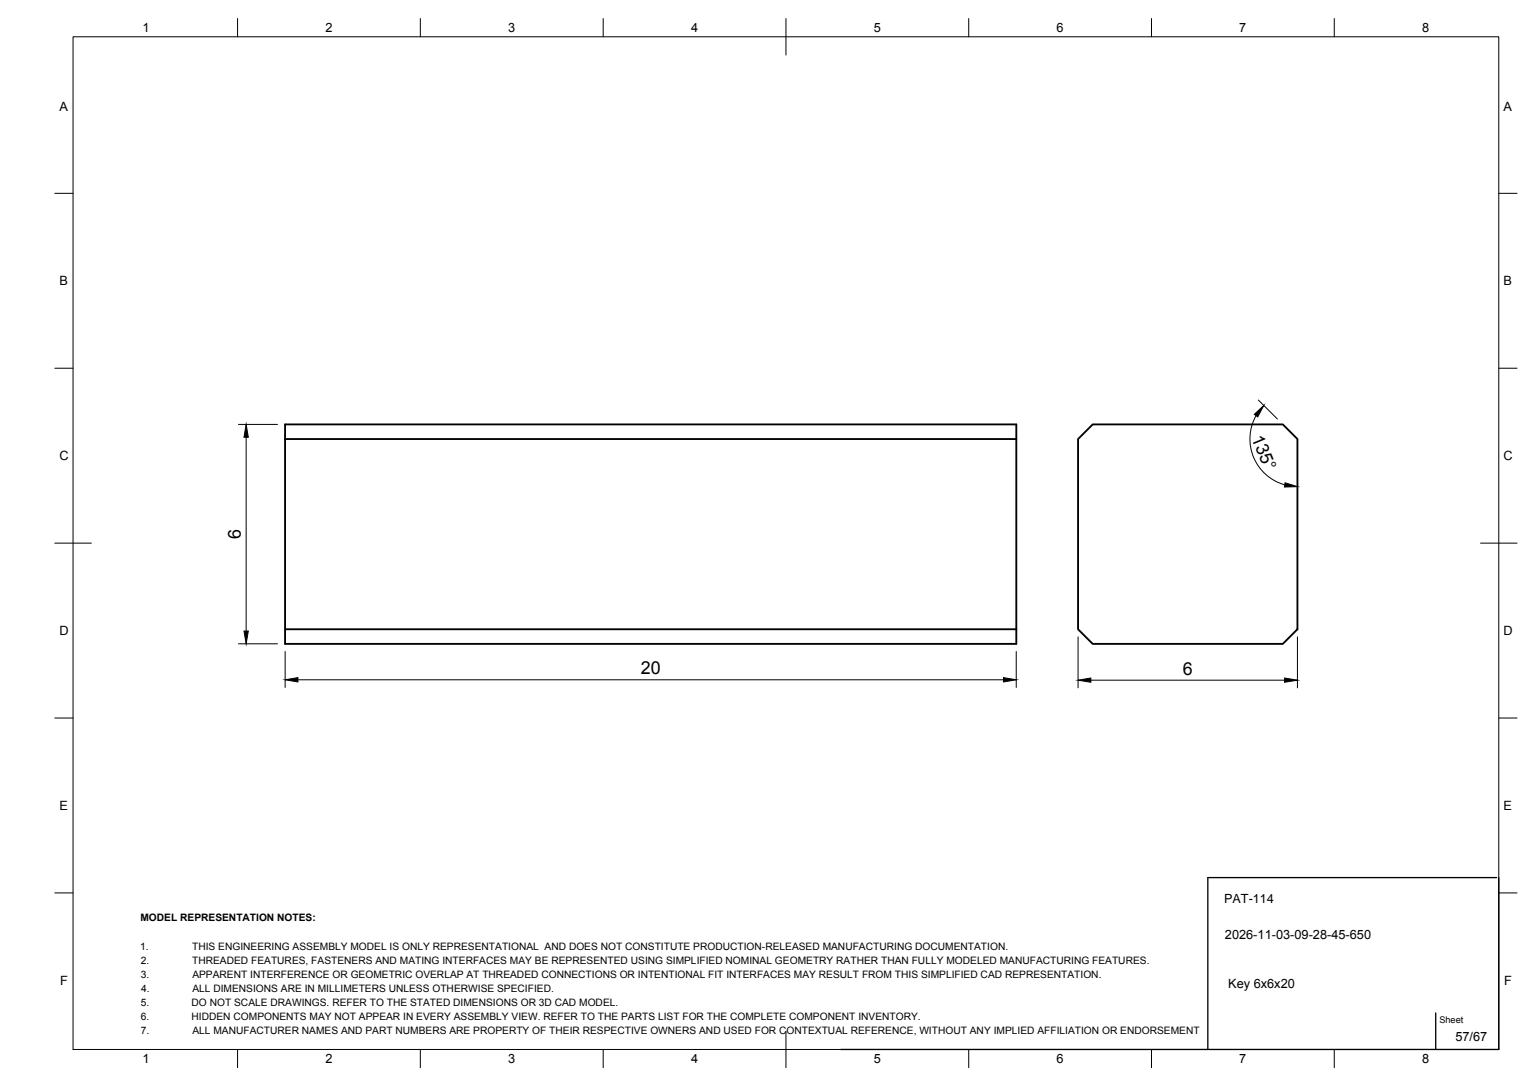
ISO-10303-21;
HEADER;
/* Generated by software containing ST-Developer
 * from STEP Tools, Inc. (www.steptools.com) 
 */

FILE_DESCRIPTION(
/* description */ ('Two-stage gear reducer in split housing'),
/* implementation_level */ '2;1');

FILE_NAME(
/* name */ 'Key 6x6x20.step',
/* time_stamp */ '2026-10-28T03:22:31-07:00',
/* author */ (''),
/* organization */ (''),
/* preprocessor_version */ 'ST-DEVELOPER v20.2',
/* originating_system */ 'Autodesk Translation Framework v15.17.0.0',
/* authorisation */ '');

FILE_SCHEMA (('AUTOMOTIVE_DESIGN { 1 0 10303 214 3 1 1 }'));
ENDSEC;

DATA;
#10=MECHANICAL_DESIGN_GEOMETRIC_PRESENTATION_REPRESENTATION('',(#1304),#73366);
#1177=SHAPE_REPRESENTATION_RELATIONSHIP('SRR','None',#73669,#1233);
#1233=ADVANCED_BREP_SHAPE_REPRESENTATION('',(#1373),#73365);
#1304=STYLED_ITEM('',(#73988),#1373);
#1373=MANIFOLD_SOLID_BREP('Body1',#16194);
#1992=PLANE('',#18419);
#1993=PLANE('',#18420);
#1994=PLANE('',#18421);
#1995=PLANE('',#18422);
#1996=PLANE('',#18423);
#1997=PLANE('',#18424);
#1998=PLANE('',#18425);
#1999=PLANE('',#18426);
#2000=PLANE('',#18427);
#2001=PLANE('',#18428);
#2905=FACE_OUTER_BOUND('',#4046,.T.);
#2906=FACE_OUTER_BOUND('',#4047,.T.);
#2907=FACE_OUTER_BOUND('',#4048,.T.);
#2908=FACE_OUTER_BOUND('',#4049,.T.);
#2909=FACE_OUTER_BOUND('',#4050,.T.);
#2910=FACE_OUTER_BOUND('',#4051,.T.);
#2911=FACE_OUTER_BOUND('',#4052,.T.);
#2912=FACE_OUTER_BOUND('',#4053,.T.);
#2913=FACE_OUTER_BOUND('',#4054,.T.);
#2914=FACE_OUTER_BOUND('',#4055,.T.);
#4046=EDGE_LOOP('',(#14859,#14860,#14861,#14862,#14863,#14864,#14865,#14866));
#4047=EDGE_LOOP('',(#14867,#14868,#14869,#14870));
#4048=EDGE_LOOP('',(#14871,#14872,#14873,#14874));
#4049=EDGE_LOOP('',(#14875,#14876,#14877,#14878));
#4050=EDGE_LOOP('',(#14879,#14880,#14881,#14882));
#4051=EDGE_LOOP('',(#14883,#14884,#14885,#14886,#14887,#14888,#14889,#14890));
#4052=EDGE_LOOP('',(#14891,#14892,#14893,#14894));
#4053=EDGE_LOOP('',(#14895,#14896,#14897,#14898));
#4054=EDGE_LOOP('',(#14899,#14900,#14901,#14902));
#4055=EDGE_LOOP('',(#14903,#14904,#14905,#14906));
#5056=LINE('',#73163,#6080);
#5057=LINE('',#73165,#6081);
#5058=LINE('',#73167,#6082);
#5059=LINE('',#73169,#6083);
#5060=LINE('',#73171,#6084);
#5061=LINE('',#73173,#6085);
#5062=LINE('',#73175,#6086);
#5063=LINE('',#73176,#6087);
#5064=LINE('',#73179,#6088);
#5065=LINE('',#73181,#6089);
#5066=LINE('',#73182,#6090);
#5067=LINE('',#73185,#6091);
#5068=LINE('',#73186,#6092);
#5069=LINE('',#73189,#6093);
#5070=LINE('',#73190,#6094);
#5071=LINE('',#73193,#6095);
#5072=LINE('',#73194,#6096);
#5073=LINE('',#73198,#6097);
#5074=LINE('',#73199,#6098);
#5075=LINE('',#73201,#6099);
#5076=LINE('',#73202,#6100);
#5077=LINE('',#73204,#6101);
#5078=LINE('',#73206,#6102);
#5079=LINE('',#73208,#6103);
#6080=VECTOR('',#22674,1.);
#6081=VECTOR('',#22675,1.);
#6082=VECTOR('',#22676,1.);
#6083=VECTOR('',#22677,1.);
#6084=VECTOR('',#22678,1.);
#6085=VECTOR('',#22679,1.);
#6086=VECTOR('',#22680,1.);
#6087=VECTOR('',#22681,1.);
#6088=VECTOR('',#22684,1.);
#6089=VECTOR('',#22685,1.);
#6090=VECTOR('',#22686,1.);
#6091=VECTOR('',#22689,1.);
#6092=VECTOR('',#22690,1.);
#6093=VECTOR('',#22693,1.);
#6094=VECTOR('',#22694,1.);
#6095=VECTOR('',#22697,1.);
#6096=VECTOR('',#22698,1.);
#6097=VECTOR('',#22701,1.);
#6098=VECTOR('',#22702,1.);
#6099=VECTOR('',#22703,1.);
#6100=VECTOR('',#22704,1.);
#6101=VECTOR('',#22707,1.);
#6102=VECTOR('',#22710,1.);
#6103=VECTOR('',#22713,1.);
#8291=VERTEX_POINT('',#73161);
#8292=VERTEX_POINT('',#73162);
#8293=VERTEX_POINT('',#73164);
#8294=VERTEX_POINT('',#73166);
#8295=VERTEX_POINT('',#73168);
#8296=VERTEX_POINT('',#73170);
#8297=VERTEX_POINT('',#73172);
#8298=VERTEX_POINT('',#73174);
#8299=VERTEX_POINT('',#73178);
#8300=VERTEX_POINT('',#73180);
#8301=VERTEX_POINT('',#73184);
#8302=VERTEX_POINT('',#73188);
#8303=VERTEX_POINT('',#73192);
#8304=VERTEX_POINT('',#73196);
#8305=VERTEX_POINT('',#73197);
#8306=VERTEX_POINT('',#73200);
#10483=EDGE_CURVE('',#8291,#8292,#5056,.T.);
#10484=EDGE_CURVE('',#8293,#8291,#5057,.T.);
#10485=EDGE_CURVE('',#8294,#8293,#5058,.T.);
#10486=EDGE_CURVE('',#8295,#8294,#5059,.T.);
#10487=EDGE_CURVE('',#8296,#8295,#5060,.T.);
#10488=EDGE_CURVE('',#8297,#8296,#5061,.T.);
#10489=EDGE_CURVE('',#8298,#8297,#5062,.T.);
#10490=EDGE_CURVE('',#8292,#8298,#5063,.T.);
#10491=EDGE_CURVE('',#8295,#8299,#5064,.T.);
#10492=EDGE_CURVE('',#8299,#8300,#5065,.T.);
#10493=EDGE_CURVE('',#8300,#8296,#5066,.T.);
#10494=EDGE_CURVE('',#8301,#8294,#5067,.T.);
#10495=EDGE_CURVE('',#8301,#8299,#5068,.T.);
#10496=EDGE_CURVE('',#8293,#8302,#5069,.T.);
#10497=EDGE_CURVE('',#8302,#8301,#5070,.T.);
#10498=EDGE_CURVE('',#8303,#8291,#5071,.T.);
#10499=EDGE_CURVE('',#8303,#8302,#5072,.T.);
#10500=EDGE_CURVE('',#8304,#8305,#5073,.T.);
#10501=EDGE_CURVE('',#8300,#8304,#5074,.T.);
#10502=EDGE_CURVE('',#8306,#8303,#5075,.T.);
#10503=EDGE_CURVE('',#8305,#8306,#5076,.T.);
#10504=EDGE_CURVE('',#8297,#8304,#5077,.T.);
#10505=EDGE_CURVE('',#8292,#8306,#5078,.T.);
#10506=EDGE_CURVE('',#8305,#8298,#5079,.T.);
#14859=ORIENTED_EDGE('',*,*,#10483,.F.);
#14860=ORIENTED_EDGE('',*,*,#10484,.F.);
#14861=ORIENTED_EDGE('',*,*,#10485,.F.);
#14862=ORIENTED_EDGE('',*,*,#10486,.F.);
#14863=ORIENTED_EDGE('',*,*,#10487,.F.);
#14864=ORIENTED_EDGE('',*,*,#10488,.F.);
#14865=ORIENTED_EDGE('',*,*,#10489,.F.);
#14866=ORIENTED_EDGE('',*,*,#10490,.F.);
#14867=ORIENTED_EDGE('',*,*,#10487,.T.);
#14868=ORIENTED_EDGE('',*,*,#10491,.T.);
#14869=ORIENTED_EDGE('',*,*,#10492,.T.);
#14870=ORIENTED_EDGE('',*,*,#10493,.T.);
#14871=ORIENTED_EDGE('',*,*,#10486,.T.);
#14872=ORIENTED_EDGE('',*,*,#10494,.F.);
#14873=ORIENTED_EDGE('',*,*,#10495,.T.);
#14874=ORIENTED_EDGE('',*,*,#10491,.F.);
#14875=ORIENTED_EDGE('',*,*,#10485,.T.);
#14876=ORIENTED_EDGE('',*,*,#10496,.T.);
#14877=ORIENTED_EDGE('',*,*,#10497,.T.);
#14878=ORIENTED_EDGE('',*,*,#10494,.T.);
#14879=ORIENTED_EDGE('',*,*,#10484,.T.);
#14880=ORIENTED_EDGE('',*,*,#10498,.F.);
#14881=ORIENTED_EDGE('',*,*,#10499,.T.);
#14882=ORIENTED_EDGE('',*,*,#10496,.F.);
#14883=ORIENTED_EDGE('',*,*,#10500,.F.);
#14884=ORIENTED_EDGE('',*,*,#10501,.F.);
#14885=ORIENTED_EDGE('',*,*,#10492,.F.);
#14886=ORIENTED_EDGE('',*,*,#10495,.F.);
#14887=ORIENTED_EDGE('',*,*,#10497,.F.);
#14888=ORIENTED_EDGE('',*,*,#10499,.F.);
#14889=ORIENTED_EDGE('',*,*,#10502,.F.);
#14890=ORIENTED_EDGE('',*,*,#10503,.F.);
#14891=ORIENTED_EDGE('',*,*,#10488,.T.);
#14892=ORIENTED_EDGE('',*,*,#10493,.F.);
#14893=ORIENTED_EDGE('',*,*,#10501,.T.);
#14894=ORIENTED_EDGE('',*,*,#10504,.F.);
#14895=ORIENTED_EDGE('',*,*,#10483,.T.);
#14896=ORIENTED_EDGE('',*,*,#10505,.T.);
#14897=ORIENTED_EDGE('',*,*,#10502,.T.);
#14898=ORIENTED_EDGE('',*,*,#10498,.T.);
#14899=ORIENTED_EDGE('',*,*,#10489,.T.);
#14900=ORIENTED_EDGE('',*,*,#10504,.T.);
#14901=ORIENTED_EDGE('',*,*,#10500,.T.);
#14902=ORIENTED_EDGE('',*,*,#10506,.T.);
#14903=ORIENTED_EDGE('',*,*,#10490,.T.);
#14904=ORIENTED_EDGE('',*,*,#10506,.F.);
#14905=ORIENTED_EDGE('',*,*,#10503,.T.);
#14906=ORIENTED_EDGE('',*,*,#10505,.F.);
#16112=ADVANCED_FACE('',(#2905),#1992,.F.);
#16113=ADVANCED_FACE('',(#2906),#1993,.T.);
#16114=ADVANCED_FACE('',(#2907),#1994,.T.);
#16115=ADVANCED_FACE('',(#2908),#1995,.T.);
#16116=ADVANCED_FACE('',(#2909),#1996,.T.);
#16117=ADVANCED_FACE('',(#2910),#1997,.T.);
#16118=ADVANCED_FACE('',(#2911),#1998,.F.);
#16119=ADVANCED_FACE('',(#2912),#1999,.T.);
#16120=ADVANCED_FACE('',(#2913),#2000,.T.);
#16121=ADVANCED_FACE('',(#2914),#2001,.T.);
#16194=CLOSED_SHELL('',(#16112,#16113,#16114,#16115,#16116,#16117,#16118,
#16119,#16120,#16121));
#18418=AXIS2_PLACEMENT_3D('',#73159,#22670,#22671);
#18419=AXIS2_PLACEMENT_3D('',#73160,#22672,#22673);
#18420=AXIS2_PLACEMENT_3D('',#73177,#22682,#22683);
#18421=AXIS2_PLACEMENT_3D('',#73183,#22687,#22688);
#18422=AXIS2_PLACEMENT_3D('',#73187,#22691,#22692);
#18423=AXIS2_PLACEMENT_3D('',#73191,#22695,#22696);
#18424=AXIS2_PLACEMENT_3D('',#73195,#22699,#22700);
#18425=AXIS2_PLACEMENT_3D('',#73203,#22705,#22706);
#18426=AXIS2_PLACEMENT_3D('',#73205,#22708,#22709);
#18427=AXIS2_PLACEMENT_3D('',#73207,#22711,#22712);
#18428=AXIS2_PLACEMENT_3D('',#73209,#22714,#22715);
#22670=DIRECTION('axis',(0.,0.,1.));
#22671=DIRECTION('refdir',(1.,0.,0.));
#22672=DIRECTION('center_axis',(1.,0.,0.));
#22673=DIRECTION('ref_axis',(0.,0.,-1.));
#22674=DIRECTION('',(0.,-0.707106781186547,-0.707106781186548));
#22675=DIRECTION('',(0.,-1.,0.));
#22676=DIRECTION('',(0.,-0.707106781186547,0.707106781186548));
#22677=DIRECTION('',(0.,0.,1.));
#22678=DIRECTION('',(0.,0.707106781186547,0.707106781186548));
#22679=DIRECTION('',(0.,1.,0.));
#22680=DIRECTION('',(0.,0.707106781186547,-0.707106781186548));
#22681=DIRECTION('',(0.,0.,-1.));
#22682=DIRECTION('center_axis',(0.,0.707106781186548,-0.707106781186547));
#22683=DIRECTION('ref_axis',(-1.,0.,0.));
#22684=DIRECTION('',(1.,0.,0.));
#22685=DIRECTION('',(0.,-0.707106781186547,-0.707106781186548));
#22686=DIRECTION('',(-1.,0.,0.));
#22687=DIRECTION('center_axis',(0.,1.,0.));
#22688=DIRECTION('ref_axis',(-1.,0.,0.));
#22689=DIRECTION('',(-1.,0.,0.));
#22690=DIRECTION('',(0.,0.,-1.));
#22691=DIRECTION('center_axis',(0.,0.707106781186548,0.707106781186547));
#22692=DIRECTION('ref_axis',(1.,0.,0.));
#22693=DIRECTION('',(1.,0.,0.));
#22694=DIRECTION('',(0.,0.707106781186547,-0.707106781186548));
#22695=DIRECTION('center_axis',(0.,0.,1.));
#22696=DIRECTION('ref_axis',(1.,0.,0.));
#22697=DIRECTION('',(-1.,0.,0.));
#22698=DIRECTION('',(0.,1.,0.));
#22699=DIRECTION('center_axis',(1.,0.,0.));
#22700=DIRECTION('ref_axis',(0.,0.,-1.));
#22701=DIRECTION('',(0.,-0.707106781186547,0.707106781186548));
#22702=DIRECTION('',(0.,-1.,0.));
#22703=DIRECTION('',(0.,0.707106781186547,0.707106781186548));
#22704=DIRECTION('',(0.,0.,1.));
#22705=DIRECTION('center_axis',(0.,0.,1.));
#22706=DIRECTION('ref_axis',(1.,0.,0.));
#22707=DIRECTION('',(1.,0.,0.));
#22708=DIRECTION('center_axis',(0.,-0.707106781186548,0.707106781186547));
#22709=DIRECTION('ref_axis',(1.,0.,0.));
#22710=DIRECTION('',(1.,0.,0.));
#22711=DIRECTION('center_axis',(0.,-0.707106781186548,-0.707106781186547));
#22712=DIRECTION('ref_axis',(-1.,0.,0.));
#22713=DIRECTION('',(-1.,0.,0.));
#22714=DIRECTION('center_axis',(0.,-1.,0.));
#22715=DIRECTION('ref_axis',(1.,0.,0.));
#73159=CARTESIAN_POINT('',(0.,0.,0.));
#73160=CARTESIAN_POINT('Origin',(-1.,0.,0.35));
#73161=CARTESIAN_POINT('',(-1.,-0.26,0.6));
#73162=CARTESIAN_POINT('',(-1.,-0.3,0.56));
#73163=CARTESIAN_POINT('',(-1.,-0.2675,0.5925));
#73164=CARTESIAN_POINT('',(-1.,0.26,0.6));
#73165=CARTESIAN_POINT('',(-1.,0.,0.6));
#73166=CARTESIAN_POINT('',(-1.,0.3,0.56));
#73167=CARTESIAN_POINT('',(-1.,0.2675,0.5925));
#73168=CARTESIAN_POINT('',(-1.,0.3,0.04));
#73169=CARTESIAN_POINT('',(-1.,0.3,0.175));
#73170=CARTESIAN_POINT('',(-1.,0.26,0.));
#73171=CARTESIAN_POINT('',(-1.,0.2925,0.0325));
#73172=CARTESIAN_POINT('',(-1.,-0.26,0.));
#73173=CARTESIAN_POINT('',(-1.,0.,0.));
#73174=CARTESIAN_POINT('',(-1.,-0.3,0.04));
#73175=CARTESIAN_POINT('',(-1.,-0.2925,0.0325));
#73176=CARTESIAN_POINT('',(-1.,-0.3,0.175));
#73177=CARTESIAN_POINT('Origin',(0.75,0.28,0.02));
#73178=CARTESIAN_POINT('',(1.,0.3,0.04));
#73179=CARTESIAN_POINT('',(0.75,0.3,0.04));
#73180=CARTESIAN_POINT('',(1.,0.26,0.));
#73181=CARTESIAN_POINT('',(1.,0.2925,0.0325));
#73182=CARTESIAN_POINT('',(0.75,0.26,0.));
#73183=CARTESIAN_POINT('Origin',(1.5,0.3,0.));
#73184=CARTESIAN_POINT('',(1.,0.3,0.56));
#73185=CARTESIAN_POINT('',(0.75,0.3,0.56));
#73186=CARTESIAN_POINT('',(1.,0.3,0.175));
#73187=CARTESIAN_POINT('Origin',(0.75,0.28,0.58));
#73188=CARTESIAN_POINT('',(1.,0.26,0.6));
#73189=CARTESIAN_POINT('',(0.75,0.26,0.6));
#73190=CARTESIAN_POINT('',(1.,0.2675,0.5925));
#73191=CARTESIAN_POINT('Origin',(0.,0.,0.6));
#73192=CARTESIAN_POINT('',(1.,-0.26,0.6));
#73193=CARTESIAN_POINT('',(-0.75,-0.26,0.6));
#73194=CARTESIAN_POINT('',(1.,0.,0.6));
#73195=CARTESIAN_POINT('Origin',(1.,0.,0.35));
#73196=CARTESIAN_POINT('',(1.,-0.26,0.));
#73197=CARTESIAN_POINT('',(1.,-0.3,0.04));
#73198=CARTESIAN_POINT('',(1.,-0.2925,0.0325));
#73199=CARTESIAN_POINT('',(1.,0.,0.));
#73200=CARTESIAN_POINT('',(1.,-0.3,0.56));
#73201=CARTESIAN_POINT('',(1.,-0.2675,0.5925));
#73202=CARTESIAN_POINT('',(1.,-0.3,0.175));
#73203=CARTESIAN_POINT('Origin',(0.,0.,0.));
#73204=CARTESIAN_POINT('',(-0.75,-0.26,0.));
#73205=CARTESIAN_POINT('Origin',(-0.75,-0.28,0.58));
#73206=CARTESIAN_POINT('',(-0.75,-0.3,0.56));
#73207=CARTESIAN_POINT('Origin',(-0.75,-0.28,0.02));
#73208=CARTESIAN_POINT('',(-0.75,-0.3,0.04));
#73209=CARTESIAN_POINT('Origin',(-1.5,-0.3,0.));
#73301=UNCERTAINTY_MEASURE_WITH_UNIT(LENGTH_MEASURE(0.001),#73367,
'DISTANCE_ACCURACY_VALUE',
'Maximum model space distance between geometric entities at asserted c
onnectivities');
#73302=UNCERTAINTY_MEASURE_WITH_UNIT(LENGTH_MEASURE(0.001),#73367,
'DISTANCE_ACCURACY_VALUE',
'Maximum model space distance between geometric entities at asserted c
onnectivities');
#73365=(
GEOMETRIC_REPRESENTATION_CONTEXT(3)
GLOBAL_UNCERTAINTY_ASSIGNED_CONTEXT((#73301))
GLOBAL_UNIT_ASSIGNED_CONTEXT((#73367,#73369,#73370))
REPRESENTATION_CONTEXT('','3D')
);
#73366=(
GEOMETRIC_REPRESENTATION_CONTEXT(3)
GLOBAL_UNCERTAINTY_ASSIGNED_CONTEXT((#73302))
GLOBAL_UNIT_ASSIGNED_CONTEXT((#73367,#73369,#73370))
REPRESENTATION_CONTEXT('','3D')
);
#73367=(
LENGTH_UNIT()
NAMED_UNIT(*)
SI_UNIT(.CENTI.,.METRE.)
);
#73369=(
NAMED_UNIT(*)
PLANE_ANGLE_UNIT()
SI_UNIT($,.RADIAN.)
);
#73370=(
NAMED_UNIT(*)
SI_UNIT($,.STERADIAN.)
SOLID_ANGLE_UNIT()
);
#73433=SHAPE_DEFINITION_REPRESENTATION(#73577,#73669);
#73577=PRODUCT_DEFINITION_SHAPE('',$,#73733);
#73669=SHAPE_REPRESENTATION('',(#18418),#73365);
#73670=PRODUCT_DEFINITION_CONTEXT('part definition',#73861,'design');
#73733=PRODUCT_DEFINITION('Key 6x6x20','Key 6x6x20',#73796,#73670);
#73796=PRODUCT_DEFINITION_FORMATION('',$,#73925);
#73861=APPLICATION_CONTEXT(
'Core Data for Automotive Mechanical Design Process');
#73862=PRODUCT_CONTEXT('part definition',#73861,'mechanical');
#73925=PRODUCT('Key 6x6x20','Key 6x6x20','Key 6x6x20',(#73862));
#73982=COLOUR_RGB('Grey',0.48,0.52,0.57);
#73983=FILL_AREA_STYLE_COLOUR('',#73982);
#73984=FILL_AREA_STYLE('',(#73983));
#73985=SURFACE_STYLE_FILL_AREA(#73984);
#73986=SURFACE_SIDE_STYLE('',(#73985));
#73987=SURFACE_STYLE_USAGE(.BOTH.,#73986);
#73988=PRESENTATION_STYLE_ASSIGNMENT((#73987));
ENDSEC;
END-ISO-10303-21;
